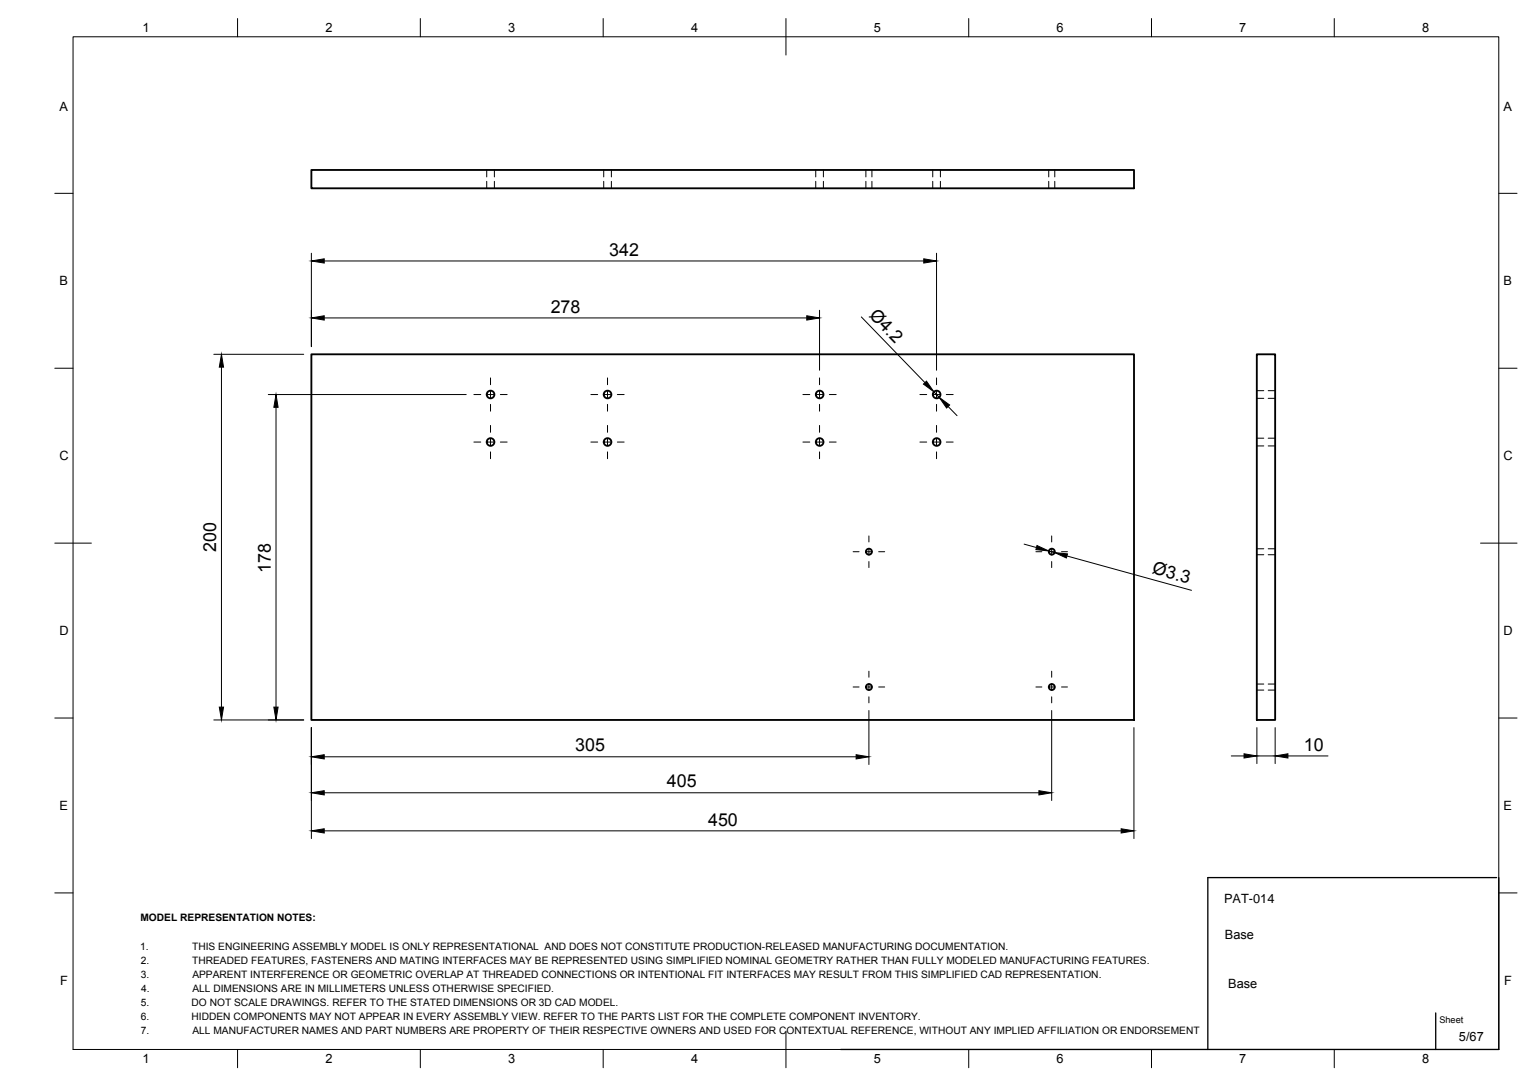
ISO-10303-21;
HEADER;
/* Generated by software containing ST-Developer
 * from STEP Tools, Inc. (www.steptools.com) 
 */

FILE_DESCRIPTION(
/* description */ ('Bin tilter linkage'),
/* implementation_level */ '2;1');

FILE_NAME(
/* name */ 'Base.step',
/* time_stamp */ '2026-10-28T03:26:24-07:00',
/* author */ (''),
/* organization */ (''),
/* preprocessor_version */ 'ST-DEVELOPER v20.2',
/* originating_system */ 'Autodesk Translation Framework v15.17.0.0',
/* authorisation */ '');

FILE_SCHEMA (('AUTOMOTIVE_DESIGN { 1 0 10303 214 3 1 1 }'));
ENDSEC;

DATA;
#10=MECHANICAL_DESIGN_GEOMETRIC_PRESENTATION_REPRESENTATION('',(#862),#23728);
#650=SHAPE_REPRESENTATION_RELATIONSHIP('SRR','None',#24114,#756);
#756=ADVANCED_BREP_SHAPE_REPRESENTATION('',(#976),#23614);
#862=STYLED_ITEM('',(#24744),#976);
#976=MANIFOLD_SOLID_BREP('Body1',#12392);
#1087=FACE_BOUND('',#2684,.T.);
#1088=FACE_BOUND('',#2685,.T.);
#1089=FACE_BOUND('',#2686,.T.);
#1090=FACE_BOUND('',#2687,.T.);
#1091=FACE_BOUND('',#2688,.T.);
#1092=FACE_BOUND('',#2689,.T.);
#1093=FACE_BOUND('',#2690,.T.);
#1094=FACE_BOUND('',#2691,.T.);
#1095=FACE_BOUND('',#2692,.T.);
#1096=FACE_BOUND('',#2693,.T.);
#1097=FACE_BOUND('',#2694,.T.);
#1098=FACE_BOUND('',#2695,.T.);
#1099=FACE_BOUND('',#2697,.T.);
#1100=FACE_BOUND('',#2698,.T.);
#1101=FACE_BOUND('',#2699,.T.);
#1102=FACE_BOUND('',#2700,.T.);
#1103=FACE_BOUND('',#2701,.T.);
#1104=FACE_BOUND('',#2702,.T.);
#1105=FACE_BOUND('',#2703,.T.);
#1106=FACE_BOUND('',#2704,.T.);
#1107=FACE_BOUND('',#2705,.T.);
#1108=FACE_BOUND('',#2706,.T.);
#1109=FACE_BOUND('',#2707,.T.);
#1110=FACE_BOUND('',#2708,.T.);
#1492=PLANE('',#13715);
#1493=PLANE('',#13716);
#1494=PLANE('',#13717);
#1495=PLANE('',#13718);
#1496=PLANE('',#13719);
#1497=PLANE('',#13720);
#1890=FACE_OUTER_BOUND('',#2667,.T.);
#1891=FACE_OUTER_BOUND('',#2668,.T.);
#1892=FACE_OUTER_BOUND('',#2669,.T.);
#1893=FACE_OUTER_BOUND('',#2670,.T.);
#1894=FACE_OUTER_BOUND('',#2671,.T.);
#1895=FACE_OUTER_BOUND('',#2672,.T.);
#1896=FACE_OUTER_BOUND('',#2673,.T.);
#1897=FACE_OUTER_BOUND('',#2674,.T.);
#1898=FACE_OUTER_BOUND('',#2675,.T.);
#1899=FACE_OUTER_BOUND('',#2676,.T.);
#1900=FACE_OUTER_BOUND('',#2677,.T.);
#1901=FACE_OUTER_BOUND('',#2678,.T.);
#1902=FACE_OUTER_BOUND('',#2679,.T.);
#1903=FACE_OUTER_BOUND('',#2680,.T.);
#1904=FACE_OUTER_BOUND('',#2681,.T.);
#1905=FACE_OUTER_BOUND('',#2682,.T.);
#1906=FACE_OUTER_BOUND('',#2683,.T.);
#1907=FACE_OUTER_BOUND('',#2696,.T.);
#2667=EDGE_LOOP('',(#8373,#8374,#8375,#8376));
#2668=EDGE_LOOP('',(#8377,#8378,#8379,#8380));
#2669=EDGE_LOOP('',(#8381,#8382,#8383,#8384));
#2670=EDGE_LOOP('',(#8385,#8386,#8387,#8388));
#2671=EDGE_LOOP('',(#8389,#8390,#8391,#8392));
#2672=EDGE_LOOP('',(#8393,#8394,#8395,#8396));
#2673=EDGE_LOOP('',(#8397,#8398,#8399,#8400));
#2674=EDGE_LOOP('',(#8401,#8402,#8403,#8404));
#2675=EDGE_LOOP('',(#8405,#8406,#8407,#8408));
#2676=EDGE_LOOP('',(#8409,#8410,#8411,#8412));
#2677=EDGE_LOOP('',(#8413,#8414,#8415,#8416));
#2678=EDGE_LOOP('',(#8417,#8418,#8419,#8420));
#2679=EDGE_LOOP('',(#8421,#8422,#8423,#8424));
#2680=EDGE_LOOP('',(#8425,#8426,#8427,#8428));
#2681=EDGE_LOOP('',(#8429,#8430,#8431,#8432));
#2682=EDGE_LOOP('',(#8433,#8434,#8435,#8436));
#2683=EDGE_LOOP('',(#8437,#8438,#8439,#8440));
#2684=EDGE_LOOP('',(#8441));
#2685=EDGE_LOOP('',(#8442));
#2686=EDGE_LOOP('',(#8443));
#2687=EDGE_LOOP('',(#8444));
#2688=EDGE_LOOP('',(#8445));
#2689=EDGE_LOOP('',(#8446));
#2690=EDGE_LOOP('',(#8447));
#2691=EDGE_LOOP('',(#8448));
#2692=EDGE_LOOP('',(#8449));
#2693=EDGE_LOOP('',(#8450));
#2694=EDGE_LOOP('',(#8451));
#2695=EDGE_LOOP('',(#8452));
#2696=EDGE_LOOP('',(#8453,#8454,#8455,#8456));
#2697=EDGE_LOOP('',(#8457));
#2698=EDGE_LOOP('',(#8458));
#2699=EDGE_LOOP('',(#8459));
#2700=EDGE_LOOP('',(#8460));
#2701=EDGE_LOOP('',(#8461));
#2702=EDGE_LOOP('',(#8462));
#2703=EDGE_LOOP('',(#8463));
#2704=EDGE_LOOP('',(#8464));
#2705=EDGE_LOOP('',(#8465));
#2706=EDGE_LOOP('',(#8466));
#2707=EDGE_LOOP('',(#8467));
#2708=EDGE_LOOP('',(#8468));
#3849=LINE('',#19752,#4524);
#3850=LINE('',#19758,#4525);
#3851=LINE('',#19764,#4526);
#3852=LINE('',#19770,#4527);
#3853=LINE('',#19776,#4528);
#3854=LINE('',#19782,#4529);
#3855=LINE('',#19788,#4530);
#3856=LINE('',#19794,#4531);
#3857=LINE('',#19800,#4532);
#3858=LINE('',#19806,#4533);
#3859=LINE('',#19812,#4534);
#3860=LINE('',#19818,#4535);
#3861=LINE('',#19823,#4536);
#3862=LINE('',#19825,#4537);
#3863=LINE('',#19827,#4538);
#3864=LINE('',#19828,#4539);
#3865=LINE('',#19831,#4540);
#3866=LINE('',#19833,#4541);
#3867=LINE('',#19834,#4542);
#3868=LINE('',#19837,#4543);
#3869=LINE('',#19839,#4544);
#3870=LINE('',#19840,#4545);
#3871=LINE('',#19842,#4546);
#3872=LINE('',#19843,#4547);
#4524=VECTOR('',#15484,0.165);
#4525=VECTOR('',#15491,0.165);
#4526=VECTOR('',#15498,0.164999999999999);
#4527=VECTOR('',#15505,0.164999999999999);
#4528=VECTOR('',#15512,0.210000000000001);
#4529=VECTOR('',#15519,0.210000000000001);
#4530=VECTOR('',#15526,0.210000000000001);
#4531=VECTOR('',#15533,0.210000000000001);
#4532=VECTOR('',#15540,0.21);
#4533=VECTOR('',#15547,0.21);
#4534=VECTOR('',#15554,0.21);
#4535=VECTOR('',#15561,0.21);
#4536=VECTOR('',#15566,1.);
#4537=VECTOR('',#15567,1.);
#4538=VECTOR('',#15568,1.);
#4539=VECTOR('',#15569,1.);
#4540=VECTOR('',#15572,1.);
#4541=VECTOR('',#15573,1.);
#4542=VECTOR('',#15574,1.);
#4543=VECTOR('',#15577,1.);
#4544=VECTOR('',#15578,1.);
#4545=VECTOR('',#15579,1.);
#4546=VECTOR('',#15582,1.);
#4547=VECTOR('',#15583,1.);
#5199=CIRCLE('',#13680,0.165);
#5200=CIRCLE('',#13681,0.165);
#5201=CIRCLE('',#13683,0.165);
#5202=CIRCLE('',#13684,0.165);
#5203=CIRCLE('',#13686,0.164999999999999);
#5204=CIRCLE('',#13687,0.164999999999999);
#5205=CIRCLE('',#13689,0.164999999999999);
#5206=CIRCLE('',#13690,0.164999999999999);
#5207=CIRCLE('',#13692,0.210000000000001);
#5208=CIRCLE('',#13693,0.210000000000001);
#5209=CIRCLE('',#13695,0.210000000000001);
#5210=CIRCLE('',#13696,0.210000000000001);
#5211=CIRCLE('',#13698,0.210000000000001);
#5212=CIRCLE('',#13699,0.210000000000001);
#5213=CIRCLE('',#13701,0.210000000000001);
#5214=CIRCLE('',#13702,0.210000000000001);
#5215=CIRCLE('',#13704,0.21);
#5216=CIRCLE('',#13705,0.21);
#5217=CIRCLE('',#13707,0.21);
#5218=CIRCLE('',#13708,0.21);
#5219=CIRCLE('',#13710,0.21);
#5220=CIRCLE('',#13711,0.21);
#5221=CIRCLE('',#13713,0.21);
#5222=CIRCLE('',#13714,0.21);
#5957=VERTEX_POINT('',#19749);
#5958=VERTEX_POINT('',#19751);
#5959=VERTEX_POINT('',#19755);
#5960=VERTEX_POINT('',#19757);
#5961=VERTEX_POINT('',#19761);
#5962=VERTEX_POINT('',#19763);
#5963=VERTEX_POINT('',#19767);
#5964=VERTEX_POINT('',#19769);
#5965=VERTEX_POINT('',#19773);
#5966=VERTEX_POINT('',#19775);
#5967=VERTEX_POINT('',#19779);
#5968=VERTEX_POINT('',#19781);
#5969=VERTEX_POINT('',#19785);
#5970=VERTEX_POINT('',#19787);
#5971=VERTEX_POINT('',#19791);
#5972=VERTEX_POINT('',#19793);
#5973=VERTEX_POINT('',#19797);
#5974=VERTEX_POINT('',#19799);
#5975=VERTEX_POINT('',#19803);
#5976=VERTEX_POINT('',#19805);
#5977=VERTEX_POINT('',#19809);
#5978=VERTEX_POINT('',#19811);
#5979=VERTEX_POINT('',#19815);
#5980=VERTEX_POINT('',#19817);
#5981=VERTEX_POINT('',#19821);
#5982=VERTEX_POINT('',#19822);
#5983=VERTEX_POINT('',#19824);
#5984=VERTEX_POINT('',#19826);
#5985=VERTEX_POINT('',#19830);
#5986=VERTEX_POINT('',#19832);
#5987=VERTEX_POINT('',#19836);
#5988=VERTEX_POINT('',#19838);
#6926=EDGE_CURVE('',#5957,#5957,#5199,.T.);
#6927=EDGE_CURVE('',#5957,#5958,#3849,.T.);
#6928=EDGE_CURVE('',#5958,#5958,#5200,.T.);
#6929=EDGE_CURVE('',#5959,#5959,#5201,.T.);
#6930=EDGE_CURVE('',#5959,#5960,#3850,.T.);
#6931=EDGE_CURVE('',#5960,#5960,#5202,.T.);
#6932=EDGE_CURVE('',#5961,#5961,#5203,.T.);
#6933=EDGE_CURVE('',#5961,#5962,#3851,.T.);
#6934=EDGE_CURVE('',#5962,#5962,#5204,.T.);
#6935=EDGE_CURVE('',#5963,#5963,#5205,.T.);
#6936=EDGE_CURVE('',#5963,#5964,#3852,.T.);
#6937=EDGE_CURVE('',#5964,#5964,#5206,.T.);
#6938=EDGE_CURVE('',#5965,#5965,#5207,.T.);
#6939=EDGE_CURVE('',#5965,#5966,#3853,.T.);
#6940=EDGE_CURVE('',#5966,#5966,#5208,.T.);
#6941=EDGE_CURVE('',#5967,#5967,#5209,.T.);
#6942=EDGE_CURVE('',#5967,#5968,#3854,.T.);
#6943=EDGE_CURVE('',#5968,#5968,#5210,.T.);
#6944=EDGE_CURVE('',#5969,#5969,#5211,.T.);
#6945=EDGE_CURVE('',#5969,#5970,#3855,.T.);
#6946=EDGE_CURVE('',#5970,#5970,#5212,.T.);
#6947=EDGE_CURVE('',#5971,#5971,#5213,.T.);
#6948=EDGE_CURVE('',#5971,#5972,#3856,.T.);
#6949=EDGE_CURVE('',#5972,#5972,#5214,.T.);
#6950=EDGE_CURVE('',#5973,#5973,#5215,.T.);
#6951=EDGE_CURVE('',#5973,#5974,#3857,.T.);
#6952=EDGE_CURVE('',#5974,#5974,#5216,.T.);
#6953=EDGE_CURVE('',#5975,#5975,#5217,.T.);
#6954=EDGE_CURVE('',#5975,#5976,#3858,.T.);
#6955=EDGE_CURVE('',#5976,#5976,#5218,.T.);
#6956=EDGE_CURVE('',#5977,#5977,#5219,.T.);
#6957=EDGE_CURVE('',#5977,#5978,#3859,.T.);
#6958=EDGE_CURVE('',#5978,#5978,#5220,.T.);
#6959=EDGE_CURVE('',#5979,#5979,#5221,.T.);
#6960=EDGE_CURVE('',#5979,#5980,#3860,.T.);
#6961=EDGE_CURVE('',#5980,#5980,#5222,.T.);
#6962=EDGE_CURVE('',#5981,#5982,#3861,.T.);
#6963=EDGE_CURVE('',#5982,#5983,#3862,.T.);
#6964=EDGE_CURVE('',#5984,#5983,#3863,.T.);
#6965=EDGE_CURVE('',#5981,#5984,#3864,.T.);
#6966=EDGE_CURVE('',#5985,#5981,#3865,.T.);
#6967=EDGE_CURVE('',#5986,#5984,#3866,.T.);
#6968=EDGE_CURVE('',#5985,#5986,#3867,.T.);
#6969=EDGE_CURVE('',#5987,#5985,#3868,.T.);
#6970=EDGE_CURVE('',#5988,#5986,#3869,.T.);
#6971=EDGE_CURVE('',#5987,#5988,#3870,.T.);
#6972=EDGE_CURVE('',#5982,#5987,#3871,.T.);
#6973=EDGE_CURVE('',#5983,#5988,#3872,.T.);
#8373=ORIENTED_EDGE('',*,*,#6926,.F.);
#8374=ORIENTED_EDGE('',*,*,#6927,.T.);
#8375=ORIENTED_EDGE('',*,*,#6928,.F.);
#8376=ORIENTED_EDGE('',*,*,#6927,.F.);
#8377=ORIENTED_EDGE('',*,*,#6929,.F.);
#8378=ORIENTED_EDGE('',*,*,#6930,.T.);
#8379=ORIENTED_EDGE('',*,*,#6931,.F.);
#8380=ORIENTED_EDGE('',*,*,#6930,.F.);
#8381=ORIENTED_EDGE('',*,*,#6932,.F.);
#8382=ORIENTED_EDGE('',*,*,#6933,.T.);
#8383=ORIENTED_EDGE('',*,*,#6934,.F.);
#8384=ORIENTED_EDGE('',*,*,#6933,.F.);
#8385=ORIENTED_EDGE('',*,*,#6935,.F.);
#8386=ORIENTED_EDGE('',*,*,#6936,.T.);
#8387=ORIENTED_EDGE('',*,*,#6937,.F.);
#8388=ORIENTED_EDGE('',*,*,#6936,.F.);
#8389=ORIENTED_EDGE('',*,*,#6938,.F.);
#8390=ORIENTED_EDGE('',*,*,#6939,.T.);
#8391=ORIENTED_EDGE('',*,*,#6940,.F.);
#8392=ORIENTED_EDGE('',*,*,#6939,.F.);
#8393=ORIENTED_EDGE('',*,*,#6941,.F.);
#8394=ORIENTED_EDGE('',*,*,#6942,.T.);
#8395=ORIENTED_EDGE('',*,*,#6943,.F.);
#8396=ORIENTED_EDGE('',*,*,#6942,.F.);
#8397=ORIENTED_EDGE('',*,*,#6944,.F.);
#8398=ORIENTED_EDGE('',*,*,#6945,.T.);
#8399=ORIENTED_EDGE('',*,*,#6946,.F.);
#8400=ORIENTED_EDGE('',*,*,#6945,.F.);
#8401=ORIENTED_EDGE('',*,*,#6947,.F.);
#8402=ORIENTED_EDGE('',*,*,#6948,.T.);
#8403=ORIENTED_EDGE('',*,*,#6949,.F.);
#8404=ORIENTED_EDGE('',*,*,#6948,.F.);
#8405=ORIENTED_EDGE('',*,*,#6950,.F.);
#8406=ORIENTED_EDGE('',*,*,#6951,.T.);
#8407=ORIENTED_EDGE('',*,*,#6952,.F.);
#8408=ORIENTED_EDGE('',*,*,#6951,.F.);
#8409=ORIENTED_EDGE('',*,*,#6953,.F.);
#8410=ORIENTED_EDGE('',*,*,#6954,.T.);
#8411=ORIENTED_EDGE('',*,*,#6955,.F.);
#8412=ORIENTED_EDGE('',*,*,#6954,.F.);
#8413=ORIENTED_EDGE('',*,*,#6956,.F.);
#8414=ORIENTED_EDGE('',*,*,#6957,.T.);
#8415=ORIENTED_EDGE('',*,*,#6958,.F.);
#8416=ORIENTED_EDGE('',*,*,#6957,.F.);
#8417=ORIENTED_EDGE('',*,*,#6959,.F.);
#8418=ORIENTED_EDGE('',*,*,#6960,.T.);
#8419=ORIENTED_EDGE('',*,*,#6961,.F.);
#8420=ORIENTED_EDGE('',*,*,#6960,.F.);
#8421=ORIENTED_EDGE('',*,*,#6962,.T.);
#8422=ORIENTED_EDGE('',*,*,#6963,.T.);
#8423=ORIENTED_EDGE('',*,*,#6964,.F.);
#8424=ORIENTED_EDGE('',*,*,#6965,.F.);
#8425=ORIENTED_EDGE('',*,*,#6966,.T.);
#8426=ORIENTED_EDGE('',*,*,#6965,.T.);
#8427=ORIENTED_EDGE('',*,*,#6967,.F.);
#8428=ORIENTED_EDGE('',*,*,#6968,.F.);
#8429=ORIENTED_EDGE('',*,*,#6969,.T.);
#8430=ORIENTED_EDGE('',*,*,#6968,.T.);
#8431=ORIENTED_EDGE('',*,*,#6970,.F.);
#8432=ORIENTED_EDGE('',*,*,#6971,.F.);
#8433=ORIENTED_EDGE('',*,*,#6972,.T.);
#8434=ORIENTED_EDGE('',*,*,#6971,.T.);
#8435=ORIENTED_EDGE('',*,*,#6973,.F.);
#8436=ORIENTED_EDGE('',*,*,#6963,.F.);
#8437=ORIENTED_EDGE('',*,*,#6973,.T.);
#8438=ORIENTED_EDGE('',*,*,#6970,.T.);
#8439=ORIENTED_EDGE('',*,*,#6967,.T.);
#8440=ORIENTED_EDGE('',*,*,#6964,.T.);
#8441=ORIENTED_EDGE('',*,*,#6931,.T.);
#8442=ORIENTED_EDGE('',*,*,#6937,.T.);
#8443=ORIENTED_EDGE('',*,*,#6961,.T.);
#8444=ORIENTED_EDGE('',*,*,#6958,.T.);
#8445=ORIENTED_EDGE('',*,*,#6955,.T.);
#8446=ORIENTED_EDGE('',*,*,#6952,.T.);
#8447=ORIENTED_EDGE('',*,*,#6949,.T.);
#8448=ORIENTED_EDGE('',*,*,#6946,.T.);
#8449=ORIENTED_EDGE('',*,*,#6943,.T.);
#8450=ORIENTED_EDGE('',*,*,#6940,.T.);
#8451=ORIENTED_EDGE('',*,*,#6934,.T.);
#8452=ORIENTED_EDGE('',*,*,#6928,.T.);
#8453=ORIENTED_EDGE('',*,*,#6972,.F.);
#8454=ORIENTED_EDGE('',*,*,#6962,.F.);
#8455=ORIENTED_EDGE('',*,*,#6966,.F.);
#8456=ORIENTED_EDGE('',*,*,#6969,.F.);
#8457=ORIENTED_EDGE('',*,*,#6929,.T.);
#8458=ORIENTED_EDGE('',*,*,#6935,.T.);
#8459=ORIENTED_EDGE('',*,*,#6959,.T.);
#8460=ORIENTED_EDGE('',*,*,#6956,.T.);
#8461=ORIENTED_EDGE('',*,*,#6953,.T.);
#8462=ORIENTED_EDGE('',*,*,#6950,.T.);
#8463=ORIENTED_EDGE('',*,*,#6947,.T.);
#8464=ORIENTED_EDGE('',*,*,#6944,.T.);
#8465=ORIENTED_EDGE('',*,*,#6941,.T.);
#8466=ORIENTED_EDGE('',*,*,#6938,.T.);
#8467=ORIENTED_EDGE('',*,*,#6932,.T.);
#8468=ORIENTED_EDGE('',*,*,#6926,.T.);
#11267=CYLINDRICAL_SURFACE('',#13679,0.165);
#11268=CYLINDRICAL_SURFACE('',#13682,0.165);
#11269=CYLINDRICAL_SURFACE('',#13685,0.164999999999999);
#11270=CYLINDRICAL_SURFACE('',#13688,0.164999999999999);
#11271=CYLINDRICAL_SURFACE('',#13691,0.210000000000001);
#11272=CYLINDRICAL_SURFACE('',#13694,0.210000000000001);
#11273=CYLINDRICAL_SURFACE('',#13697,0.210000000000001);
#11274=CYLINDRICAL_SURFACE('',#13700,0.210000000000001);
#11275=CYLINDRICAL_SURFACE('',#13703,0.21);
#11276=CYLINDRICAL_SURFACE('',#13706,0.21);
#11277=CYLINDRICAL_SURFACE('',#13709,0.21);
#11278=CYLINDRICAL_SURFACE('',#13712,0.21);
#11615=ADVANCED_FACE('',(#1890),#11267,.F.);
#11616=ADVANCED_FACE('',(#1891),#11268,.F.);
#11617=ADVANCED_FACE('',(#1892),#11269,.F.);
#11618=ADVANCED_FACE('',(#1893),#11270,.F.);
#11619=ADVANCED_FACE('',(#1894),#11271,.F.);
#11620=ADVANCED_FACE('',(#1895),#11272,.F.);
#11621=ADVANCED_FACE('',(#1896),#11273,.F.);
#11622=ADVANCED_FACE('',(#1897),#11274,.F.);
#11623=ADVANCED_FACE('',(#1898),#11275,.F.);
#11624=ADVANCED_FACE('',(#1899),#11276,.F.);
#11625=ADVANCED_FACE('',(#1900),#11277,.F.);
#11626=ADVANCED_FACE('',(#1901),#11278,.F.);
#11627=ADVANCED_FACE('',(#1902),#1492,.T.);
#11628=ADVANCED_FACE('',(#1903),#1493,.T.);
#11629=ADVANCED_FACE('',(#1904),#1494,.T.);
#11630=ADVANCED_FACE('',(#1905),#1495,.T.);
#11631=ADVANCED_FACE('',(#1906,#1087,#1088,#1089,#1090,#1091,#1092,#1093,
#1094,#1095,#1096,#1097,#1098),#1496,.T.);
#11632=ADVANCED_FACE('',(#1907,#1099,#1100,#1101,#1102,#1103,#1104,#1105,
#1106,#1107,#1108,#1109,#1110),#1497,.F.);
#12392=CLOSED_SHELL('',(#11615,#11616,#11617,#11618,#11619,#11620,#11621,
#11622,#11623,#11624,#11625,#11626,#11627,#11628,#11629,#11630,#11631,#11632));
#13678=AXIS2_PLACEMENT_3D('',#19747,#15478,#15479);
#13679=AXIS2_PLACEMENT_3D('',#19748,#15480,#15481);
#13680=AXIS2_PLACEMENT_3D('',#19750,#15482,#15483);
#13681=AXIS2_PLACEMENT_3D('',#19753,#15485,#15486);
#13682=AXIS2_PLACEMENT_3D('',#19754,#15487,#15488);
#13683=AXIS2_PLACEMENT_3D('',#19756,#15489,#15490);
#13684=AXIS2_PLACEMENT_3D('',#19759,#15492,#15493);
#13685=AXIS2_PLACEMENT_3D('',#19760,#15494,#15495);
#13686=AXIS2_PLACEMENT_3D('',#19762,#15496,#15497);
#13687=AXIS2_PLACEMENT_3D('',#19765,#15499,#15500);
#13688=AXIS2_PLACEMENT_3D('',#19766,#15501,#15502);
#13689=AXIS2_PLACEMENT_3D('',#19768,#15503,#15504);
#13690=AXIS2_PLACEMENT_3D('',#19771,#15506,#15507);
#13691=AXIS2_PLACEMENT_3D('',#19772,#15508,#15509);
#13692=AXIS2_PLACEMENT_3D('',#19774,#15510,#15511);
#13693=AXIS2_PLACEMENT_3D('',#19777,#15513,#15514);
#13694=AXIS2_PLACEMENT_3D('',#19778,#15515,#15516);
#13695=AXIS2_PLACEMENT_3D('',#19780,#15517,#15518);
#13696=AXIS2_PLACEMENT_3D('',#19783,#15520,#15521);
#13697=AXIS2_PLACEMENT_3D('',#19784,#15522,#15523);
#13698=AXIS2_PLACEMENT_3D('',#19786,#15524,#15525);
#13699=AXIS2_PLACEMENT_3D('',#19789,#15527,#15528);
#13700=AXIS2_PLACEMENT_3D('',#19790,#15529,#15530);
#13701=AXIS2_PLACEMENT_3D('',#19792,#15531,#15532);
#13702=AXIS2_PLACEMENT_3D('',#19795,#15534,#15535);
#13703=AXIS2_PLACEMENT_3D('',#19796,#15536,#15537);
#13704=AXIS2_PLACEMENT_3D('',#19798,#15538,#15539);
#13705=AXIS2_PLACEMENT_3D('',#19801,#15541,#15542);
#13706=AXIS2_PLACEMENT_3D('',#19802,#15543,#15544);
#13707=AXIS2_PLACEMENT_3D('',#19804,#15545,#15546);
#13708=AXIS2_PLACEMENT_3D('',#19807,#15548,#15549);
#13709=AXIS2_PLACEMENT_3D('',#19808,#15550,#15551);
#13710=AXIS2_PLACEMENT_3D('',#19810,#15552,#15553);
#13711=AXIS2_PLACEMENT_3D('',#19813,#15555,#15556);
#13712=AXIS2_PLACEMENT_3D('',#19814,#15557,#15558);
#13713=AXIS2_PLACEMENT_3D('',#19816,#15559,#15560);
#13714=AXIS2_PLACEMENT_3D('',#19819,#15562,#15563);
#13715=AXIS2_PLACEMENT_3D('',#19820,#15564,#15565);
#13716=AXIS2_PLACEMENT_3D('',#19829,#15570,#15571);
#13717=AXIS2_PLACEMENT_3D('',#19835,#15575,#15576);
#13718=AXIS2_PLACEMENT_3D('',#19841,#15580,#15581);
#13719=AXIS2_PLACEMENT_3D('',#19844,#15584,#15585);
#13720=AXIS2_PLACEMENT_3D('',#19845,#15586,#15587);
#15478=DIRECTION('axis',(0.,0.,1.));
#15479=DIRECTION('refdir',(1.,0.,0.));
#15480=DIRECTION('center_axis',(0.,0.,1.));
#15481=DIRECTION('ref_axis',(1.,0.,0.));
#15482=DIRECTION('center_axis',(0.,0.,1.));
#15483=DIRECTION('ref_axis',(1.,0.,0.));
#15484=DIRECTION('',(0.,0.,1.));
#15485=DIRECTION('center_axis',(0.,0.,-1.));
#15486=DIRECTION('ref_axis',(1.,0.,0.));
#15487=DIRECTION('center_axis',(0.,0.,1.));
#15488=DIRECTION('ref_axis',(1.,0.,0.));
#15489=DIRECTION('center_axis',(0.,0.,1.));
#15490=DIRECTION('ref_axis',(1.,0.,0.));
#15491=DIRECTION('',(0.,0.,1.));
#15492=DIRECTION('center_axis',(0.,0.,-1.));
#15493=DIRECTION('ref_axis',(1.,0.,0.));
#15494=DIRECTION('center_axis',(0.,0.,1.));
#15495=DIRECTION('ref_axis',(1.,0.,0.));
#15496=DIRECTION('center_axis',(0.,0.,1.));
#15497=DIRECTION('ref_axis',(1.,0.,0.));
#15498=DIRECTION('',(0.,0.,1.));
#15499=DIRECTION('center_axis',(0.,0.,-1.));
#15500=DIRECTION('ref_axis',(1.,0.,0.));
#15501=DIRECTION('center_axis',(0.,0.,1.));
#15502=DIRECTION('ref_axis',(1.,0.,0.));
#15503=DIRECTION('center_axis',(0.,0.,1.));
#15504=DIRECTION('ref_axis',(1.,0.,0.));
#15505=DIRECTION('',(0.,0.,1.));
#15506=DIRECTION('center_axis',(0.,0.,-1.));
#15507=DIRECTION('ref_axis',(1.,0.,0.));
#15508=DIRECTION('center_axis',(0.,0.,1.));
#15509=DIRECTION('ref_axis',(1.,0.,0.));
#15510=DIRECTION('center_axis',(0.,0.,1.));
#15511=DIRECTION('ref_axis',(1.,0.,0.));
#15512=DIRECTION('',(0.,0.,1.));
#15513=DIRECTION('center_axis',(0.,0.,-1.));
#15514=DIRECTION('ref_axis',(1.,0.,0.));
#15515=DIRECTION('center_axis',(0.,0.,1.));
#15516=DIRECTION('ref_axis',(1.,0.,0.));
#15517=DIRECTION('center_axis',(0.,0.,1.));
#15518=DIRECTION('ref_axis',(1.,0.,0.));
#15519=DIRECTION('',(0.,0.,1.));
#15520=DIRECTION('center_axis',(0.,0.,-1.));
#15521=DIRECTION('ref_axis',(1.,0.,0.));
#15522=DIRECTION('center_axis',(0.,0.,1.));
#15523=DIRECTION('ref_axis',(1.,0.,0.));
#15524=DIRECTION('center_axis',(0.,0.,1.));
#15525=DIRECTION('ref_axis',(1.,0.,0.));
#15526=DIRECTION('',(0.,0.,1.));
#15527=DIRECTION('center_axis',(0.,0.,-1.));
#15528=DIRECTION('ref_axis',(1.,0.,0.));
#15529=DIRECTION('center_axis',(0.,0.,1.));
#15530=DIRECTION('ref_axis',(1.,0.,0.));
#15531=DIRECTION('center_axis',(0.,0.,1.));
#15532=DIRECTION('ref_axis',(1.,0.,0.));
#15533=DIRECTION('',(0.,0.,1.));
#15534=DIRECTION('center_axis',(0.,0.,-1.));
#15535=DIRECTION('ref_axis',(1.,0.,0.));
#15536=DIRECTION('center_axis',(0.,0.,1.));
#15537=DIRECTION('ref_axis',(1.,0.,0.));
#15538=DIRECTION('center_axis',(0.,0.,1.));
#15539=DIRECTION('ref_axis',(1.,0.,0.));
#15540=DIRECTION('',(0.,0.,1.));
#15541=DIRECTION('center_axis',(0.,0.,-1.));
#15542=DIRECTION('ref_axis',(1.,0.,0.));
#15543=DIRECTION('center_axis',(0.,0.,1.));
#15544=DIRECTION('ref_axis',(1.,0.,0.));
#15545=DIRECTION('center_axis',(0.,0.,1.));
#15546=DIRECTION('ref_axis',(1.,0.,0.));
#15547=DIRECTION('',(0.,0.,1.));
#15548=DIRECTION('center_axis',(0.,0.,-1.));
#15549=DIRECTION('ref_axis',(1.,0.,0.));
#15550=DIRECTION('center_axis',(0.,0.,1.));
#15551=DIRECTION('ref_axis',(1.,0.,0.));
#15552=DIRECTION('center_axis',(0.,0.,1.));
#15553=DIRECTION('ref_axis',(1.,0.,0.));
#15554=DIRECTION('',(0.,0.,1.));
#15555=DIRECTION('center_axis',(0.,0.,-1.));
#15556=DIRECTION('ref_axis',(1.,0.,0.));
#15557=DIRECTION('center_axis',(0.,0.,1.));
#15558=DIRECTION('ref_axis',(1.,0.,0.));
#15559=DIRECTION('center_axis',(0.,0.,1.));
#15560=DIRECTION('ref_axis',(1.,0.,0.));
#15561=DIRECTION('',(0.,0.,1.));
#15562=DIRECTION('center_axis',(0.,0.,-1.));
#15563=DIRECTION('ref_axis',(1.,0.,0.));
#15564=DIRECTION('center_axis',(0.,1.,0.));
#15565=DIRECTION('ref_axis',(-1.,0.,0.));
#15566=DIRECTION('',(-1.,0.,0.));
#15567=DIRECTION('',(0.,0.,1.));
#15568=DIRECTION('',(-1.,0.,0.));
#15569=DIRECTION('',(0.,0.,1.));
#15570=DIRECTION('center_axis',(1.,0.,0.));
#15571=DIRECTION('ref_axis',(0.,1.,0.));
#15572=DIRECTION('',(0.,1.,0.));
#15573=DIRECTION('',(0.,1.,0.));
#15574=DIRECTION('',(0.,0.,1.));
#15575=DIRECTION('center_axis',(0.,-1.,0.));
#15576=DIRECTION('ref_axis',(1.,0.,0.));
#15577=DIRECTION('',(1.,0.,0.));
#15578=DIRECTION('',(1.,0.,0.));
#15579=DIRECTION('',(0.,0.,1.));
#15580=DIRECTION('center_axis',(-1.,0.,0.));
#15581=DIRECTION('ref_axis',(0.,-1.,0.));
#15582=DIRECTION('',(0.,-1.,0.));
#15583=DIRECTION('',(0.,-1.,0.));
#15584=DIRECTION('center_axis',(0.,0.,1.));
#15585=DIRECTION('ref_axis',(1.,0.,0.));
#15586=DIRECTION('center_axis',(0.,0.,1.));
#15587=DIRECTION('ref_axis',(1.,0.,0.));
#19747=CARTESIAN_POINT('',(0.,0.,0.));
#19748=CARTESIAN_POINT('Origin',(0.5,-0.8,-0.1));
#19749=CARTESIAN_POINT('',(0.335,-0.8,0.));
#19750=CARTESIAN_POINT('Origin',(0.5,-0.8,0.));
#19751=CARTESIAN_POINT('',(0.335,-0.8,1.));
#19752=CARTESIAN_POINT('',(0.335,-0.8,-0.1));
#19753=CARTESIAN_POINT('Origin',(0.5,-0.8,1.));
#19754=CARTESIAN_POINT('Origin',(0.5,-8.2,-0.1));
#19755=CARTESIAN_POINT('',(0.335,-8.2,0.));
#19756=CARTESIAN_POINT('Origin',(0.5,-8.2,0.));
#19757=CARTESIAN_POINT('',(0.335,-8.2,1.));
#19758=CARTESIAN_POINT('',(0.335,-8.2,-0.1));
#19759=CARTESIAN_POINT('Origin',(0.5,-8.2,1.));
#19760=CARTESIAN_POINT('Origin',(-9.5,-0.8,-0.1));
#19761=CARTESIAN_POINT('',(-9.665,-0.8,0.));
#19762=CARTESIAN_POINT('Origin',(-9.5,-0.8,0.));
#19763=CARTESIAN_POINT('',(-9.665,-0.8,1.));
#19764=CARTESIAN_POINT('',(-9.665,-0.8,-0.1));
#19765=CARTESIAN_POINT('Origin',(-9.5,-0.8,1.));
#19766=CARTESIAN_POINT('Origin',(-9.5,-8.2,-0.1));
#19767=CARTESIAN_POINT('',(-9.665,-8.2,0.));
#19768=CARTESIAN_POINT('Origin',(-9.5,-8.2,0.));
#19769=CARTESIAN_POINT('',(-9.665,-8.2,1.));
#19770=CARTESIAN_POINT('',(-9.665,-8.2,-0.1));
#19771=CARTESIAN_POINT('Origin',(-9.5,-8.2,1.));
#19772=CARTESIAN_POINT('Origin',(21.2,7.8,-0.1));
#19773=CARTESIAN_POINT('',(20.99,7.8,0.));
#19774=CARTESIAN_POINT('Origin',(21.2,7.8,0.));
#19775=CARTESIAN_POINT('',(20.99,7.8,1.));
#19776=CARTESIAN_POINT('',(20.99,7.8,-0.1));
#19777=CARTESIAN_POINT('Origin',(21.2,7.8,1.));
#19778=CARTESIAN_POINT('Origin',(21.2,5.2,-0.1));
#19779=CARTESIAN_POINT('',(20.99,5.2,0.));
#19780=CARTESIAN_POINT('Origin',(21.2,5.2,0.));
#19781=CARTESIAN_POINT('',(20.99,5.2,1.));
#19782=CARTESIAN_POINT('',(20.99,5.2,-0.1));
#19783=CARTESIAN_POINT('Origin',(21.2,5.2,1.));
#19784=CARTESIAN_POINT('Origin',(14.8,7.8,-0.1));
#19785=CARTESIAN_POINT('',(14.59,7.8,0.));
#19786=CARTESIAN_POINT('Origin',(14.8,7.8,0.));
#19787=CARTESIAN_POINT('',(14.59,7.8,1.));
#19788=CARTESIAN_POINT('',(14.59,7.8,-0.1));
#19789=CARTESIAN_POINT('Origin',(14.8,7.8,1.));
#19790=CARTESIAN_POINT('Origin',(14.8,5.2,-0.1));
#19791=CARTESIAN_POINT('',(14.59,5.2,0.));
#19792=CARTESIAN_POINT('Origin',(14.8,5.2,0.));
#19793=CARTESIAN_POINT('',(14.59,5.2,1.));
#19794=CARTESIAN_POINT('',(14.59,5.2,-0.1));
#19795=CARTESIAN_POINT('Origin',(14.8,5.2,1.));
#19796=CARTESIAN_POINT('Origin',(3.2,7.8,-0.1));
#19797=CARTESIAN_POINT('',(2.99,7.8,0.));
#19798=CARTESIAN_POINT('Origin',(3.2,7.8,0.));
#19799=CARTESIAN_POINT('',(2.99,7.8,1.));
#19800=CARTESIAN_POINT('',(2.99,7.8,-0.1));
#19801=CARTESIAN_POINT('Origin',(3.2,7.8,1.));
#19802=CARTESIAN_POINT('Origin',(3.2,5.2,-0.1));
#19803=CARTESIAN_POINT('',(2.99,5.2,0.));
#19804=CARTESIAN_POINT('Origin',(3.2,5.2,0.));
#19805=CARTESIAN_POINT('',(2.99,5.2,1.));
#19806=CARTESIAN_POINT('',(2.99,5.2,-0.1));
#19807=CARTESIAN_POINT('Origin',(3.2,5.2,1.));
#19808=CARTESIAN_POINT('Origin',(-3.2,7.8,-0.1));
#19809=CARTESIAN_POINT('',(-3.41,7.8,0.));
#19810=CARTESIAN_POINT('Origin',(-3.2,7.8,0.));
#19811=CARTESIAN_POINT('',(-3.41,7.8,1.));
#19812=CARTESIAN_POINT('',(-3.41,7.8,-0.1));
#19813=CARTESIAN_POINT('Origin',(-3.2,7.8,1.));
#19814=CARTESIAN_POINT('Origin',(-3.2,5.2,-0.1));
#19815=CARTESIAN_POINT('',(-3.41,5.2,0.));
#19816=CARTESIAN_POINT('Origin',(-3.2,5.2,0.));
#19817=CARTESIAN_POINT('',(-3.41,5.2,1.));
#19818=CARTESIAN_POINT('',(-3.41,5.2,-0.1));
#19819=CARTESIAN_POINT('Origin',(-3.2,5.2,1.));
#19820=CARTESIAN_POINT('Origin',(31.,10.,0.));
#19821=CARTESIAN_POINT('',(31.,10.,0.));
#19822=CARTESIAN_POINT('',(-14.,10.,0.));
#19823=CARTESIAN_POINT('',(31.,10.,0.));
#19824=CARTESIAN_POINT('',(-14.,10.,1.));
#19825=CARTESIAN_POINT('',(-14.,10.,0.));
#19826=CARTESIAN_POINT('',(31.,10.,1.));
#19827=CARTESIAN_POINT('',(31.,10.,1.));
#19828=CARTESIAN_POINT('',(31.,10.,0.));
#19829=CARTESIAN_POINT('Origin',(31.,-10.,0.));
#19830=CARTESIAN_POINT('',(31.,-10.,0.));
#19831=CARTESIAN_POINT('',(31.,-10.,0.));
#19832=CARTESIAN_POINT('',(31.,-10.,1.));
#19833=CARTESIAN_POINT('',(31.,-10.,1.));
#19834=CARTESIAN_POINT('',(31.,-10.,0.));
#19835=CARTESIAN_POINT('Origin',(-14.,-10.,0.));
#19836=CARTESIAN_POINT('',(-14.,-10.,0.));
#19837=CARTESIAN_POINT('',(-14.,-10.,0.));
#19838=CARTESIAN_POINT('',(-14.,-10.,1.));
#19839=CARTESIAN_POINT('',(-14.,-10.,1.));
#19840=CARTESIAN_POINT('',(-14.,-10.,0.));
#19841=CARTESIAN_POINT('Origin',(-14.,10.,0.));
#19842=CARTESIAN_POINT('',(-14.,10.,0.));
#19843=CARTESIAN_POINT('',(-14.,10.,1.));
#19844=CARTESIAN_POINT('Origin',(8.5,0.,1.));
#19845=CARTESIAN_POINT('Origin',(8.5,0.,0.));
#23497=UNCERTAINTY_MEASURE_WITH_UNIT(LENGTH_MEASURE(0.001),#23729,
'DISTANCE_ACCURACY_VALUE',
'Maximum model space distance between geometric entities at asserted c
onnectivities');
#23611=UNCERTAINTY_MEASURE_WITH_UNIT(LENGTH_MEASURE(0.001),#23729,
'DISTANCE_ACCURACY_VALUE',
'Maximum model space distance between geometric entities at asserted c
onnectivities');
#23614=(
GEOMETRIC_REPRESENTATION_CONTEXT(3)
GLOBAL_UNCERTAINTY_ASSIGNED_CONTEXT((#23497))
GLOBAL_UNIT_ASSIGNED_CONTEXT((#23729,#23731,#23732))
REPRESENTATION_CONTEXT('','3D')
);
#23728=(
GEOMETRIC_REPRESENTATION_CONTEXT(3)
GLOBAL_UNCERTAINTY_ASSIGNED_CONTEXT((#23611))
GLOBAL_UNIT_ASSIGNED_CONTEXT((#23729,#23731,#23732))
REPRESENTATION_CONTEXT('','3D')
);
#23729=(
LENGTH_UNIT()
NAMED_UNIT(*)
SI_UNIT(.CENTI.,.METRE.)
);
#23731=(
NAMED_UNIT(*)
PLANE_ANGLE_UNIT()
SI_UNIT($,.RADIAN.)
);
#23732=(
NAMED_UNIT(*)
SI_UNIT($,.STERADIAN.)
SOLID_ANGLE_UNIT()
);
#23735=SHAPE_DEFINITION_REPRESENTATION(#23851,#24114);
#23851=PRODUCT_DEFINITION_SHAPE('',$,#24231);
#24114=SHAPE_REPRESENTATION('',(#13678),#23614);
#24228=PRODUCT_DEFINITION_CONTEXT('part definition',#24578,'design');
#24231=PRODUCT_DEFINITION('Base','Base',#24347,#24228);
#24347=PRODUCT_DEFINITION_FORMATION('',$,#24582);
#24578=APPLICATION_CONTEXT(
'Core Data for Automotive Mechanical Design Process');
#24579=PRODUCT_CONTEXT('part definition',#24578,'mechanical');
#24582=PRODUCT('Base','Base','Base',(#24579));
#24738=COLOUR_RGB('Dark Blue',0.08,0.2,0.34);
#24739=FILL_AREA_STYLE_COLOUR('',#24738);
#24740=FILL_AREA_STYLE('',(#24739));
#24741=SURFACE_STYLE_FILL_AREA(#24740);
#24742=SURFACE_SIDE_STYLE('',(#24741));
#24743=SURFACE_STYLE_USAGE(.BOTH.,#24742);
#24744=PRESENTATION_STYLE_ASSIGNMENT((#24743));
ENDSEC;
END-ISO-10303-21;
